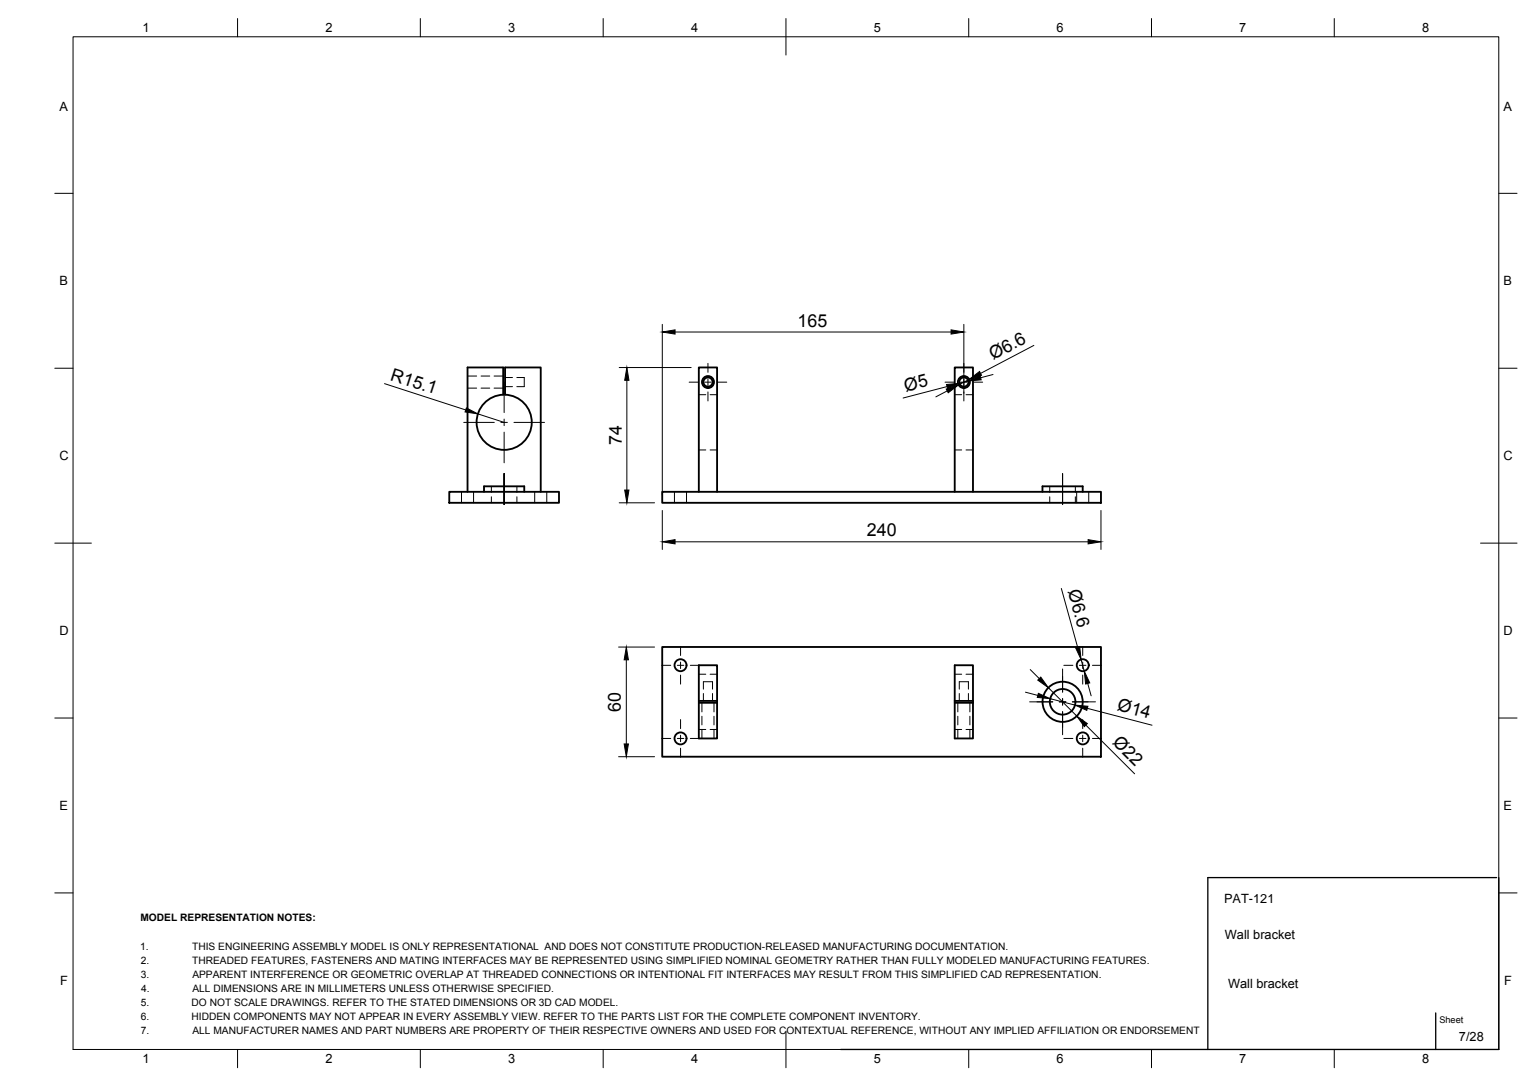
ISO-10303-21;
HEADER;
/* Generated by software containing ST-Developer
 * from STEP Tools, Inc. (www.steptools.com) 
 */

FILE_DESCRIPTION(
/* description */ ('Wall-mounted air drop station'),
/* implementation_level */ '2;1');

FILE_NAME(
/* name */ 'Wall bracket.step',
/* time_stamp */ '2026-10-28T22:16:19-07:00',
/* author */ (''),
/* organization */ (''),
/* preprocessor_version */ 'ST-DEVELOPER v20.2',
/* originating_system */ 'Autodesk Translation Framework v15.17.0.0',
/* authorisation */ '');

FILE_SCHEMA (('AUTOMOTIVE_DESIGN { 1 0 10303 214 3 1 1 }'));
ENDSEC;

DATA;
#10=MECHANICAL_DESIGN_GEOMETRIC_PRESENTATION_REPRESENTATION('',(#346),#10517);
#288=SHAPE_REPRESENTATION_RELATIONSHIP('SRR','None',#10645,#317);
#317=ADVANCED_BREP_SHAPE_REPRESENTATION('',(#375),#10489);
#346=STYLED_ITEM('',(#10853),#375);
#375=MANIFOLD_SOLID_BREP('Body1',#5885);
#407=FACE_BOUND('',#1141,.T.);
#408=FACE_BOUND('',#1146,.T.);
#409=FACE_BOUND('',#1148,.T.);
#410=FACE_BOUND('',#1155,.T.);
#411=FACE_BOUND('',#1161,.T.);
#412=FACE_BOUND('',#1163,.T.);
#413=FACE_BOUND('',#1170,.T.);
#414=FACE_BOUND('',#1174,.T.);
#415=FACE_BOUND('',#1175,.T.);
#416=FACE_BOUND('',#1176,.T.);
#417=FACE_BOUND('',#1177,.T.);
#418=FACE_BOUND('',#1178,.T.);
#419=FACE_BOUND('',#1179,.T.);
#420=FACE_BOUND('',#1180,.T.);
#421=FACE_BOUND('',#1183,.T.);
#422=FACE_BOUND('',#1184,.T.);
#423=FACE_BOUND('',#1185,.T.);
#424=FACE_BOUND('',#1186,.T.);
#425=FACE_BOUND('',#1187,.T.);
#534=PLANE('',#6290);
#535=PLANE('',#6294);
#536=PLANE('',#6298);
#537=PLANE('',#6299);
#538=PLANE('',#6300);
#539=PLANE('',#6304);
#540=PLANE('',#6305);
#541=PLANE('',#6306);
#542=PLANE('',#6307);
#543=PLANE('',#6308);
#544=PLANE('',#6312);
#545=PLANE('',#6316);
#546=PLANE('',#6317);
#547=PLANE('',#6318);
#548=PLANE('',#6322);
#549=PLANE('',#6323);
#550=PLANE('',#6324);
#551=PLANE('',#6325);
#552=PLANE('',#6326);
#553=PLANE('',#6327);
#554=PLANE('',#6328);
#555=PLANE('',#6329);
#556=PLANE('',#6330);
#557=PLANE('',#6331);
#558=PLANE('',#6332);
#771=FACE_OUTER_BOUND('',#1134,.T.);
#772=FACE_OUTER_BOUND('',#1135,.T.);
#773=FACE_OUTER_BOUND('',#1136,.T.);
#774=FACE_OUTER_BOUND('',#1137,.T.);
#775=FACE_OUTER_BOUND('',#1138,.T.);
#776=FACE_OUTER_BOUND('',#1139,.T.);
#777=FACE_OUTER_BOUND('',#1140,.T.);
#778=FACE_OUTER_BOUND('',#1142,.T.);
#779=FACE_OUTER_BOUND('',#1143,.T.);
#780=FACE_OUTER_BOUND('',#1144,.T.);
#781=FACE_OUTER_BOUND('',#1145,.T.);
#782=FACE_OUTER_BOUND('',#1147,.T.);
#783=FACE_OUTER_BOUND('',#1149,.T.);
#784=FACE_OUTER_BOUND('',#1150,.T.);
#785=FACE_OUTER_BOUND('',#1151,.T.);
#786=FACE_OUTER_BOUND('',#1152,.T.);
#787=FACE_OUTER_BOUND('',#1153,.T.);
#788=FACE_OUTER_BOUND('',#1154,.T.);
#789=FACE_OUTER_BOUND('',#1156,.T.);
#790=FACE_OUTER_BOUND('',#1157,.T.);
#791=FACE_OUTER_BOUND('',#1158,.T.);
#792=FACE_OUTER_BOUND('',#1159,.T.);
#793=FACE_OUTER_BOUND('',#1160,.T.);
#794=FACE_OUTER_BOUND('',#1162,.T.);
#795=FACE_OUTER_BOUND('',#1164,.T.);
#796=FACE_OUTER_BOUND('',#1165,.T.);
#797=FACE_OUTER_BOUND('',#1166,.T.);
#798=FACE_OUTER_BOUND('',#1167,.T.);
#799=FACE_OUTER_BOUND('',#1168,.T.);
#800=FACE_OUTER_BOUND('',#1169,.T.);
#801=FACE_OUTER_BOUND('',#1171,.T.);
#802=FACE_OUTER_BOUND('',#1172,.T.);
#803=FACE_OUTER_BOUND('',#1173,.T.);
#804=FACE_OUTER_BOUND('',#1181,.T.);
#805=FACE_OUTER_BOUND('',#1182,.T.);
#806=FACE_OUTER_BOUND('',#1188,.T.);
#807=FACE_OUTER_BOUND('',#1189,.T.);
#1134=EDGE_LOOP('',(#4021,#4022,#4023,#4024));
#1135=EDGE_LOOP('',(#4025,#4026,#4027,#4028));
#1136=EDGE_LOOP('',(#4029,#4030,#4031,#4032));
#1137=EDGE_LOOP('',(#4033,#4034,#4035,#4036));
#1138=EDGE_LOOP('',(#4037,#4038,#4039,#4040));
#1139=EDGE_LOOP('',(#4041,#4042,#4043,#4044));
#1140=EDGE_LOOP('',(#4045));
#1141=EDGE_LOOP('',(#4046));
#1142=EDGE_LOOP('',(#4047,#4048,#4049,#4050));
#1143=EDGE_LOOP('',(#4051));
#1144=EDGE_LOOP('',(#4052,#4053,#4054,#4055));
#1145=EDGE_LOOP('',(#4056,#4057,#4058,#4059));
#1146=EDGE_LOOP('',(#4060));
#1147=EDGE_LOOP('',(#4061,#4062,#4063,#4064));
#1148=EDGE_LOOP('',(#4065));
#1149=EDGE_LOOP('',(#4066,#4067,#4068,#4069,#4070,#4071,#4072,#4073));
#1150=EDGE_LOOP('',(#4074,#4075,#4076,#4077));
#1151=EDGE_LOOP('',(#4078,#4079,#4080,#4081));
#1152=EDGE_LOOP('',(#4082,#4083,#4084,#4085));
#1153=EDGE_LOOP('',(#4086,#4087,#4088,#4089));
#1154=EDGE_LOOP('',(#4090,#4091,#4092,#4093));
#1155=EDGE_LOOP('',(#4094));
#1156=EDGE_LOOP('',(#4095,#4096,#4097,#4098,#4099,#4100,#4101,#4102));
#1157=EDGE_LOOP('',(#4103,#4104,#4105,#4106));
#1158=EDGE_LOOP('',(#4107));
#1159=EDGE_LOOP('',(#4108,#4109,#4110,#4111));
#1160=EDGE_LOOP('',(#4112,#4113,#4114,#4115));
#1161=EDGE_LOOP('',(#4116));
#1162=EDGE_LOOP('',(#4117,#4118,#4119,#4120));
#1163=EDGE_LOOP('',(#4121));
#1164=EDGE_LOOP('',(#4122,#4123,#4124,#4125,#4126,#4127,#4128,#4129));
#1165=EDGE_LOOP('',(#4130,#4131,#4132,#4133));
#1166=EDGE_LOOP('',(#4134,#4135,#4136,#4137));
#1167=EDGE_LOOP('',(#4138,#4139,#4140,#4141));
#1168=EDGE_LOOP('',(#4142,#4143,#4144,#4145));
#1169=EDGE_LOOP('',(#4146,#4147,#4148,#4149));
#1170=EDGE_LOOP('',(#4150));
#1171=EDGE_LOOP('',(#4151,#4152,#4153,#4154,#4155,#4156,#4157,#4158));
#1172=EDGE_LOOP('',(#4159,#4160,#4161,#4162));
#1173=EDGE_LOOP('',(#4163,#4164,#4165,#4166));
#1174=EDGE_LOOP('',(#4167,#4168,#4169,#4170));
#1175=EDGE_LOOP('',(#4171,#4172,#4173,#4174));
#1176=EDGE_LOOP('',(#4175));
#1177=EDGE_LOOP('',(#4176));
#1178=EDGE_LOOP('',(#4177));
#1179=EDGE_LOOP('',(#4178));
#1180=EDGE_LOOP('',(#4179));
#1181=EDGE_LOOP('',(#4180,#4181,#4182,#4183));
#1182=EDGE_LOOP('',(#4184,#4185,#4186,#4187));
#1183=EDGE_LOOP('',(#4188));
#1184=EDGE_LOOP('',(#4189));
#1185=EDGE_LOOP('',(#4190));
#1186=EDGE_LOOP('',(#4191));
#1187=EDGE_LOOP('',(#4192));
#1188=EDGE_LOOP('',(#4193,#4194,#4195,#4196));
#1189=EDGE_LOOP('',(#4197,#4198,#4199,#4200));
#1600=LINE('',#8831,#2064);
#1601=LINE('',#8837,#2065);
#1602=LINE('',#8843,#2066);
#1603=LINE('',#8849,#2067);
#1604=LINE('',#8855,#2068);
#1605=LINE('',#8861,#2069);
#1606=LINE('',#8868,#2070);
#1607=LINE('',#8875,#2071);
#1608=LINE('',#8880,#2072);
#1609=LINE('',#8882,#2073);
#1610=LINE('',#8884,#2074);
#1611=LINE('',#8885,#2075);
#1612=LINE('',#8889,#2076);
#1613=LINE('',#8891,#2077);
#1614=LINE('',#8893,#2078);
#1615=LINE('',#8894,#2079);
#1616=LINE('',#8897,#2080);
#1617=LINE('',#8899,#2081);
#1618=LINE('',#8901,#2082);
#1619=LINE('',#8903,#2083);
#1620=LINE('',#8904,#2084);
#1621=LINE('',#8910,#2085);
#1622=LINE('',#8911,#2086);
#1623=LINE('',#8915,#2087);
#1624=LINE('',#8916,#2088);
#1625=LINE('',#8917,#2089);
#1626=LINE('',#8919,#2090);
#1627=LINE('',#8922,#2091);
#1628=LINE('',#8923,#2092);
#1629=LINE('',#8925,#2093);
#1630=LINE('',#8930,#2094);
#1631=LINE('',#8937,#2095);
#1632=LINE('',#8942,#2096);
#1633=LINE('',#8944,#2097);
#1634=LINE('',#8946,#2098);
#1635=LINE('',#8947,#2099);
#1636=LINE('',#8951,#2100);
#1637=LINE('',#8953,#2101);
#1638=LINE('',#8955,#2102);
#1639=LINE('',#8956,#2103);
#1640=LINE('',#8959,#2104);
#1641=LINE('',#8961,#2105);
#1642=LINE('',#8963,#2106);
#1643=LINE('',#8965,#2107);
#1644=LINE('',#8966,#2108);
#1645=LINE('',#8972,#2109);
#1646=LINE('',#8973,#2110);
#1647=LINE('',#8977,#2111);
#1648=LINE('',#8978,#2112);
#1649=LINE('',#8979,#2113);
#1650=LINE('',#8981,#2114);
#1651=LINE('',#8984,#2115);
#1652=LINE('',#8985,#2116);
#1653=LINE('',#8987,#2117);
#1654=LINE('',#8991,#2118);
#1655=LINE('',#8993,#2119);
#1656=LINE('',#8995,#2120);
#1657=LINE('',#8996,#2121);
#1658=LINE('',#8999,#2122);
#1659=LINE('',#9001,#2123);
#1660=LINE('',#9002,#2124);
#1661=LINE('',#9005,#2125);
#1662=LINE('',#9007,#2126);
#1663=LINE('',#9008,#2127);
#1664=LINE('',#9010,#2128);
#1665=LINE('',#9011,#2129);
#2064=VECTOR('',#7010,0.33);
#2065=VECTOR('',#7017,0.33);
#2066=VECTOR('',#7024,0.33);
#2067=VECTOR('',#7031,0.33);
#2068=VECTOR('',#7038,0.7);
#2069=VECTOR('',#7045,1.1);
#2070=VECTOR('',#7054,0.25);
#2071=VECTOR('',#7063,0.33);
#2072=VECTOR('',#7068,1.);
#2073=VECTOR('',#7069,1.);
#2074=VECTOR('',#7070,1.);
#2075=VECTOR('',#7071,1.);
#2076=VECTOR('',#7074,1.);
#2077=VECTOR('',#7075,1.);
#2078=VECTOR('',#7076,1.);
#2079=VECTOR('',#7077,1.);
#2080=VECTOR('',#7080,1.);
#2081=VECTOR('',#7081,1.);
#2082=VECTOR('',#7082,1.);
#2083=VECTOR('',#7083,1.);
#2084=VECTOR('',#7084,1.);
#2085=VECTOR('',#7093,1.);
#2086=VECTOR('',#7094,1.);
#2087=VECTOR('',#7097,1.);
#2088=VECTOR('',#7098,1.);
#2089=VECTOR('',#7099,1.);
#2090=VECTOR('',#7102,1.);
#2091=VECTOR('',#7105,1.);
#2092=VECTOR('',#7106,1.);
#2093=VECTOR('',#7109,1.);
#2094=VECTOR('',#7114,0.25);
#2095=VECTOR('',#7123,0.33);
#2096=VECTOR('',#7128,1.);
#2097=VECTOR('',#7129,1.);
#2098=VECTOR('',#7130,1.);
#2099=VECTOR('',#7131,1.);
#2100=VECTOR('',#7134,1.);
#2101=VECTOR('',#7135,1.);
#2102=VECTOR('',#7136,1.);
#2103=VECTOR('',#7137,1.);
#2104=VECTOR('',#7140,1.);
#2105=VECTOR('',#7141,1.);
#2106=VECTOR('',#7142,1.);
#2107=VECTOR('',#7143,1.);
#2108=VECTOR('',#7144,1.);
#2109=VECTOR('',#7153,1.);
#2110=VECTOR('',#7154,1.);
#2111=VECTOR('',#7157,1.);
#2112=VECTOR('',#7158,1.);
#2113=VECTOR('',#7159,1.);
#2114=VECTOR('',#7162,1.);
#2115=VECTOR('',#7165,1.);
#2116=VECTOR('',#7166,1.);
#2117=VECTOR('',#7169,1.);
#2118=VECTOR('',#7172,1.);
#2119=VECTOR('',#7173,1.);
#2120=VECTOR('',#7174,1.);
#2121=VECTOR('',#7175,1.);
#2122=VECTOR('',#7178,1.);
#2123=VECTOR('',#7179,1.);
#2124=VECTOR('',#7180,1.);
#2125=VECTOR('',#7183,1.);
#2126=VECTOR('',#7184,1.);
#2127=VECTOR('',#7185,1.);
#2128=VECTOR('',#7188,1.);
#2129=VECTOR('',#7189,1.);
#2536=CIRCLE('',#6273,0.33);
#2537=CIRCLE('',#6274,0.33);
#2538=CIRCLE('',#6276,0.33);
#2539=CIRCLE('',#6277,0.33);
#2540=CIRCLE('',#6279,0.33);
#2541=CIRCLE('',#6280,0.33);
#2542=CIRCLE('',#6282,0.33);
#2543=CIRCLE('',#6283,0.33);
#2544=CIRCLE('',#6285,0.7);
#2545=CIRCLE('',#6286,0.7);
#2546=CIRCLE('',#6288,1.1);
#2547=CIRCLE('',#6289,1.1);
#2548=CIRCLE('',#6292,0.25);
#2549=CIRCLE('',#6293,0.25);
#2550=CIRCLE('',#6296,0.33);
#2551=CIRCLE('',#6297,0.33);
#2552=CIRCLE('',#6301,1.51);
#2553=CIRCLE('',#6303,1.51);
#2554=CIRCLE('',#6310,0.25);
#2555=CIRCLE('',#6311,0.25);
#2556=CIRCLE('',#6314,0.33);
#2557=CIRCLE('',#6315,0.33);
#2558=CIRCLE('',#6319,1.51);
#2559=CIRCLE('',#6321,1.51);
#2781=VERTEX_POINT('',#8828);
#2782=VERTEX_POINT('',#8830);
#2783=VERTEX_POINT('',#8834);
#2784=VERTEX_POINT('',#8836);
#2785=VERTEX_POINT('',#8840);
#2786=VERTEX_POINT('',#8842);
#2787=VERTEX_POINT('',#8846);
#2788=VERTEX_POINT('',#8848);
#2789=VERTEX_POINT('',#8852);
#2790=VERTEX_POINT('',#8854);
#2791=VERTEX_POINT('',#8858);
#2792=VERTEX_POINT('',#8860);
#2793=VERTEX_POINT('',#8865);
#2794=VERTEX_POINT('',#8867);
#2795=VERTEX_POINT('',#8872);
#2796=VERTEX_POINT('',#8874);
#2797=VERTEX_POINT('',#8878);
#2798=VERTEX_POINT('',#8879);
#2799=VERTEX_POINT('',#8881);
#2800=VERTEX_POINT('',#8883);
#2801=VERTEX_POINT('',#8887);
#2802=VERTEX_POINT('',#8888);
#2803=VERTEX_POINT('',#8890);
#2804=VERTEX_POINT('',#8892);
#2805=VERTEX_POINT('',#8896);
#2806=VERTEX_POINT('',#8898);
#2807=VERTEX_POINT('',#8900);
#2808=VERTEX_POINT('',#8902);
#2809=VERTEX_POINT('',#8909);
#2810=VERTEX_POINT('',#8913);
#2811=VERTEX_POINT('',#8914);
#2812=VERTEX_POINT('',#8921);
#2813=VERTEX_POINT('',#8927);
#2814=VERTEX_POINT('',#8929);
#2815=VERTEX_POINT('',#8934);
#2816=VERTEX_POINT('',#8936);
#2817=VERTEX_POINT('',#8940);
#2818=VERTEX_POINT('',#8941);
#2819=VERTEX_POINT('',#8943);
#2820=VERTEX_POINT('',#8945);
#2821=VERTEX_POINT('',#8949);
#2822=VERTEX_POINT('',#8950);
#2823=VERTEX_POINT('',#8952);
#2824=VERTEX_POINT('',#8954);
#2825=VERTEX_POINT('',#8958);
#2826=VERTEX_POINT('',#8960);
#2827=VERTEX_POINT('',#8962);
#2828=VERTEX_POINT('',#8964);
#2829=VERTEX_POINT('',#8971);
#2830=VERTEX_POINT('',#8975);
#2831=VERTEX_POINT('',#8976);
#2832=VERTEX_POINT('',#8983);
#2833=VERTEX_POINT('',#8989);
#2834=VERTEX_POINT('',#8990);
#2835=VERTEX_POINT('',#8992);
#2836=VERTEX_POINT('',#8994);
#2837=VERTEX_POINT('',#8998);
#2838=VERTEX_POINT('',#9000);
#2839=VERTEX_POINT('',#9004);
#2840=VERTEX_POINT('',#9006);
#3268=EDGE_CURVE('',#2781,#2781,#2536,.T.);
#3269=EDGE_CURVE('',#2781,#2782,#1600,.T.);
#3270=EDGE_CURVE('',#2782,#2782,#2537,.T.);
#3271=EDGE_CURVE('',#2783,#2783,#2538,.T.);
#3272=EDGE_CURVE('',#2783,#2784,#1601,.T.);
#3273=EDGE_CURVE('',#2784,#2784,#2539,.T.);
#3274=EDGE_CURVE('',#2785,#2785,#2540,.T.);
#3275=EDGE_CURVE('',#2785,#2786,#1602,.T.);
#3276=EDGE_CURVE('',#2786,#2786,#2541,.T.);
#3277=EDGE_CURVE('',#2787,#2787,#2542,.T.);
#3278=EDGE_CURVE('',#2787,#2788,#1603,.T.);
#3279=EDGE_CURVE('',#2788,#2788,#2543,.T.);
#3280=EDGE_CURVE('',#2789,#2789,#2544,.T.);
#3281=EDGE_CURVE('',#2789,#2790,#1604,.T.);
#3282=EDGE_CURVE('',#2790,#2790,#2545,.T.);
#3283=EDGE_CURVE('',#2791,#2791,#2546,.T.);
#3284=EDGE_CURVE('',#2791,#2792,#1605,.T.);
#3285=EDGE_CURVE('',#2792,#2792,#2547,.T.);
#3286=EDGE_CURVE('',#2793,#2793,#2548,.T.);
#3287=EDGE_CURVE('',#2793,#2794,#1606,.T.);
#3288=EDGE_CURVE('',#2794,#2794,#2549,.T.);
#3289=EDGE_CURVE('',#2795,#2795,#2550,.T.);
#3290=EDGE_CURVE('',#2795,#2796,#1607,.T.);
#3291=EDGE_CURVE('',#2796,#2796,#2551,.T.);
#3292=EDGE_CURVE('',#2797,#2798,#1608,.T.);
#3293=EDGE_CURVE('',#2799,#2797,#1609,.T.);
#3294=EDGE_CURVE('',#2800,#2799,#1610,.T.);
#3295=EDGE_CURVE('',#2798,#2800,#1611,.T.);
#3296=EDGE_CURVE('',#2801,#2802,#1612,.T.);
#3297=EDGE_CURVE('',#2803,#2801,#1613,.T.);
#3298=EDGE_CURVE('',#2804,#2803,#1614,.T.);
#3299=EDGE_CURVE('',#2802,#2804,#1615,.T.);
#3300=EDGE_CURVE('',#2797,#2805,#1616,.T.);
#3301=EDGE_CURVE('',#2805,#2806,#1617,.T.);
#3302=EDGE_CURVE('',#2807,#2806,#1618,.T.);
#3303=EDGE_CURVE('',#2807,#2808,#1619,.T.);
#3304=EDGE_CURVE('',#2808,#2802,#1620,.T.);
#3305=EDGE_CURVE('',#2804,#2799,#2552,.T.);
#3306=EDGE_CURVE('',#2800,#2803,#2553,.T.);
#3307=EDGE_CURVE('',#2809,#2808,#1621,.T.);
#3308=EDGE_CURVE('',#2801,#2809,#1622,.T.);
#3309=EDGE_CURVE('',#2810,#2811,#1623,.T.);
#3310=EDGE_CURVE('',#2806,#2810,#1624,.T.);
#3311=EDGE_CURVE('',#2811,#2805,#1625,.T.);
#3312=EDGE_CURVE('',#2811,#2798,#1626,.T.);
#3313=EDGE_CURVE('',#2809,#2812,#1627,.T.);
#3314=EDGE_CURVE('',#2812,#2807,#1628,.T.);
#3315=EDGE_CURVE('',#2810,#2812,#1629,.T.);
#3316=EDGE_CURVE('',#2813,#2813,#2554,.T.);
#3317=EDGE_CURVE('',#2813,#2814,#1630,.T.);
#3318=EDGE_CURVE('',#2814,#2814,#2555,.T.);
#3319=EDGE_CURVE('',#2815,#2815,#2556,.T.);
#3320=EDGE_CURVE('',#2815,#2816,#1631,.T.);
#3321=EDGE_CURVE('',#2816,#2816,#2557,.T.);
#3322=EDGE_CURVE('',#2817,#2818,#1632,.T.);
#3323=EDGE_CURVE('',#2819,#2817,#1633,.T.);
#3324=EDGE_CURVE('',#2820,#2819,#1634,.T.);
#3325=EDGE_CURVE('',#2818,#2820,#1635,.T.);
#3326=EDGE_CURVE('',#2821,#2822,#1636,.T.);
#3327=EDGE_CURVE('',#2823,#2821,#1637,.T.);
#3328=EDGE_CURVE('',#2824,#2823,#1638,.T.);
#3329=EDGE_CURVE('',#2822,#2824,#1639,.T.);
#3330=EDGE_CURVE('',#2817,#2825,#1640,.T.);
#3331=EDGE_CURVE('',#2825,#2826,#1641,.T.);
#3332=EDGE_CURVE('',#2827,#2826,#1642,.T.);
#3333=EDGE_CURVE('',#2827,#2828,#1643,.T.);
#3334=EDGE_CURVE('',#2828,#2822,#1644,.T.);
#3335=EDGE_CURVE('',#2824,#2819,#2558,.T.);
#3336=EDGE_CURVE('',#2820,#2823,#2559,.T.);
#3337=EDGE_CURVE('',#2829,#2828,#1645,.T.);
#3338=EDGE_CURVE('',#2821,#2829,#1646,.T.);
#3339=EDGE_CURVE('',#2830,#2831,#1647,.T.);
#3340=EDGE_CURVE('',#2826,#2830,#1648,.T.);
#3341=EDGE_CURVE('',#2831,#2825,#1649,.T.);
#3342=EDGE_CURVE('',#2831,#2818,#1650,.T.);
#3343=EDGE_CURVE('',#2829,#2832,#1651,.T.);
#3344=EDGE_CURVE('',#2832,#2827,#1652,.T.);
#3345=EDGE_CURVE('',#2830,#2832,#1653,.T.);
#3346=EDGE_CURVE('',#2833,#2834,#1654,.T.);
#3347=EDGE_CURVE('',#2834,#2835,#1655,.T.);
#3348=EDGE_CURVE('',#2836,#2835,#1656,.T.);
#3349=EDGE_CURVE('',#2833,#2836,#1657,.T.);
#3350=EDGE_CURVE('',#2837,#2833,#1658,.T.);
#3351=EDGE_CURVE('',#2838,#2836,#1659,.T.);
#3352=EDGE_CURVE('',#2837,#2838,#1660,.T.);
#3353=EDGE_CURVE('',#2839,#2837,#1661,.T.);
#3354=EDGE_CURVE('',#2840,#2838,#1662,.T.);
#3355=EDGE_CURVE('',#2839,#2840,#1663,.T.);
#3356=EDGE_CURVE('',#2834,#2839,#1664,.T.);
#3357=EDGE_CURVE('',#2835,#2840,#1665,.T.);
#4021=ORIENTED_EDGE('',*,*,#3268,.F.);
#4022=ORIENTED_EDGE('',*,*,#3269,.T.);
#4023=ORIENTED_EDGE('',*,*,#3270,.F.);
#4024=ORIENTED_EDGE('',*,*,#3269,.F.);
#4025=ORIENTED_EDGE('',*,*,#3271,.F.);
#4026=ORIENTED_EDGE('',*,*,#3272,.T.);
#4027=ORIENTED_EDGE('',*,*,#3273,.F.);
#4028=ORIENTED_EDGE('',*,*,#3272,.F.);
#4029=ORIENTED_EDGE('',*,*,#3274,.F.);
#4030=ORIENTED_EDGE('',*,*,#3275,.T.);
#4031=ORIENTED_EDGE('',*,*,#3276,.F.);
#4032=ORIENTED_EDGE('',*,*,#3275,.F.);
#4033=ORIENTED_EDGE('',*,*,#3277,.F.);
#4034=ORIENTED_EDGE('',*,*,#3278,.T.);
#4035=ORIENTED_EDGE('',*,*,#3279,.F.);
#4036=ORIENTED_EDGE('',*,*,#3278,.F.);
#4037=ORIENTED_EDGE('',*,*,#3280,.F.);
#4038=ORIENTED_EDGE('',*,*,#3281,.T.);
#4039=ORIENTED_EDGE('',*,*,#3282,.F.);
#4040=ORIENTED_EDGE('',*,*,#3281,.F.);
#4041=ORIENTED_EDGE('',*,*,#3283,.F.);
#4042=ORIENTED_EDGE('',*,*,#3284,.T.);
#4043=ORIENTED_EDGE('',*,*,#3285,.F.);
#4044=ORIENTED_EDGE('',*,*,#3284,.F.);
#4045=ORIENTED_EDGE('',*,*,#3283,.T.);
#4046=ORIENTED_EDGE('',*,*,#3282,.T.);
#4047=ORIENTED_EDGE('',*,*,#3286,.F.);
#4048=ORIENTED_EDGE('',*,*,#3287,.T.);
#4049=ORIENTED_EDGE('',*,*,#3288,.F.);
#4050=ORIENTED_EDGE('',*,*,#3287,.F.);
#4051=ORIENTED_EDGE('',*,*,#3286,.T.);
#4052=ORIENTED_EDGE('',*,*,#3289,.F.);
#4053=ORIENTED_EDGE('',*,*,#3290,.T.);
#4054=ORIENTED_EDGE('',*,*,#3291,.F.);
#4055=ORIENTED_EDGE('',*,*,#3290,.F.);
#4056=ORIENTED_EDGE('',*,*,#3292,.F.);
#4057=ORIENTED_EDGE('',*,*,#3293,.F.);
#4058=ORIENTED_EDGE('',*,*,#3294,.F.);
#4059=ORIENTED_EDGE('',*,*,#3295,.F.);
#4060=ORIENTED_EDGE('',*,*,#3288,.T.);
#4061=ORIENTED_EDGE('',*,*,#3296,.F.);
#4062=ORIENTED_EDGE('',*,*,#3297,.F.);
#4063=ORIENTED_EDGE('',*,*,#3298,.F.);
#4064=ORIENTED_EDGE('',*,*,#3299,.F.);
#4065=ORIENTED_EDGE('',*,*,#3289,.T.);
#4066=ORIENTED_EDGE('',*,*,#3293,.T.);
#4067=ORIENTED_EDGE('',*,*,#3300,.T.);
#4068=ORIENTED_EDGE('',*,*,#3301,.T.);
#4069=ORIENTED_EDGE('',*,*,#3302,.F.);
#4070=ORIENTED_EDGE('',*,*,#3303,.T.);
#4071=ORIENTED_EDGE('',*,*,#3304,.T.);
#4072=ORIENTED_EDGE('',*,*,#3299,.T.);
#4073=ORIENTED_EDGE('',*,*,#3305,.T.);
#4074=ORIENTED_EDGE('',*,*,#3294,.T.);
#4075=ORIENTED_EDGE('',*,*,#3305,.F.);
#4076=ORIENTED_EDGE('',*,*,#3298,.T.);
#4077=ORIENTED_EDGE('',*,*,#3306,.F.);
#4078=ORIENTED_EDGE('',*,*,#3296,.T.);
#4079=ORIENTED_EDGE('',*,*,#3304,.F.);
#4080=ORIENTED_EDGE('',*,*,#3307,.F.);
#4081=ORIENTED_EDGE('',*,*,#3308,.F.);
#4082=ORIENTED_EDGE('',*,*,#3309,.F.);
#4083=ORIENTED_EDGE('',*,*,#3310,.F.);
#4084=ORIENTED_EDGE('',*,*,#3301,.F.);
#4085=ORIENTED_EDGE('',*,*,#3311,.F.);
#4086=ORIENTED_EDGE('',*,*,#3292,.T.);
#4087=ORIENTED_EDGE('',*,*,#3312,.F.);
#4088=ORIENTED_EDGE('',*,*,#3311,.T.);
#4089=ORIENTED_EDGE('',*,*,#3300,.F.);
#4090=ORIENTED_EDGE('',*,*,#3313,.F.);
#4091=ORIENTED_EDGE('',*,*,#3307,.T.);
#4092=ORIENTED_EDGE('',*,*,#3303,.F.);
#4093=ORIENTED_EDGE('',*,*,#3314,.F.);
#4094=ORIENTED_EDGE('',*,*,#3291,.T.);
#4095=ORIENTED_EDGE('',*,*,#3295,.T.);
#4096=ORIENTED_EDGE('',*,*,#3306,.T.);
#4097=ORIENTED_EDGE('',*,*,#3297,.T.);
#4098=ORIENTED_EDGE('',*,*,#3308,.T.);
#4099=ORIENTED_EDGE('',*,*,#3313,.T.);
#4100=ORIENTED_EDGE('',*,*,#3315,.F.);
#4101=ORIENTED_EDGE('',*,*,#3309,.T.);
#4102=ORIENTED_EDGE('',*,*,#3312,.T.);
#4103=ORIENTED_EDGE('',*,*,#3316,.F.);
#4104=ORIENTED_EDGE('',*,*,#3317,.T.);
#4105=ORIENTED_EDGE('',*,*,#3318,.F.);
#4106=ORIENTED_EDGE('',*,*,#3317,.F.);
#4107=ORIENTED_EDGE('',*,*,#3316,.T.);
#4108=ORIENTED_EDGE('',*,*,#3319,.F.);
#4109=ORIENTED_EDGE('',*,*,#3320,.T.);
#4110=ORIENTED_EDGE('',*,*,#3321,.F.);
#4111=ORIENTED_EDGE('',*,*,#3320,.F.);
#4112=ORIENTED_EDGE('',*,*,#3322,.F.);
#4113=ORIENTED_EDGE('',*,*,#3323,.F.);
#4114=ORIENTED_EDGE('',*,*,#3324,.F.);
#4115=ORIENTED_EDGE('',*,*,#3325,.F.);
#4116=ORIENTED_EDGE('',*,*,#3318,.T.);
#4117=ORIENTED_EDGE('',*,*,#3326,.F.);
#4118=ORIENTED_EDGE('',*,*,#3327,.F.);
#4119=ORIENTED_EDGE('',*,*,#3328,.F.);
#4120=ORIENTED_EDGE('',*,*,#3329,.F.);
#4121=ORIENTED_EDGE('',*,*,#3319,.T.);
#4122=ORIENTED_EDGE('',*,*,#3323,.T.);
#4123=ORIENTED_EDGE('',*,*,#3330,.T.);
#4124=ORIENTED_EDGE('',*,*,#3331,.T.);
#4125=ORIENTED_EDGE('',*,*,#3332,.F.);
#4126=ORIENTED_EDGE('',*,*,#3333,.T.);
#4127=ORIENTED_EDGE('',*,*,#3334,.T.);
#4128=ORIENTED_EDGE('',*,*,#3329,.T.);
#4129=ORIENTED_EDGE('',*,*,#3335,.T.);
#4130=ORIENTED_EDGE('',*,*,#3324,.T.);
#4131=ORIENTED_EDGE('',*,*,#3335,.F.);
#4132=ORIENTED_EDGE('',*,*,#3328,.T.);
#4133=ORIENTED_EDGE('',*,*,#3336,.F.);
#4134=ORIENTED_EDGE('',*,*,#3326,.T.);
#4135=ORIENTED_EDGE('',*,*,#3334,.F.);
#4136=ORIENTED_EDGE('',*,*,#3337,.F.);
#4137=ORIENTED_EDGE('',*,*,#3338,.F.);
#4138=ORIENTED_EDGE('',*,*,#3339,.F.);
#4139=ORIENTED_EDGE('',*,*,#3340,.F.);
#4140=ORIENTED_EDGE('',*,*,#3331,.F.);
#4141=ORIENTED_EDGE('',*,*,#3341,.F.);
#4142=ORIENTED_EDGE('',*,*,#3322,.T.);
#4143=ORIENTED_EDGE('',*,*,#3342,.F.);
#4144=ORIENTED_EDGE('',*,*,#3341,.T.);
#4145=ORIENTED_EDGE('',*,*,#3330,.F.);
#4146=ORIENTED_EDGE('',*,*,#3343,.F.);
#4147=ORIENTED_EDGE('',*,*,#3337,.T.);
#4148=ORIENTED_EDGE('',*,*,#3333,.F.);
#4149=ORIENTED_EDGE('',*,*,#3344,.F.);
#4150=ORIENTED_EDGE('',*,*,#3321,.T.);
#4151=ORIENTED_EDGE('',*,*,#3325,.T.);
#4152=ORIENTED_EDGE('',*,*,#3336,.T.);
#4153=ORIENTED_EDGE('',*,*,#3327,.T.);
#4154=ORIENTED_EDGE('',*,*,#3338,.T.);
#4155=ORIENTED_EDGE('',*,*,#3343,.T.);
#4156=ORIENTED_EDGE('',*,*,#3345,.F.);
#4157=ORIENTED_EDGE('',*,*,#3339,.T.);
#4158=ORIENTED_EDGE('',*,*,#3342,.T.);
#4159=ORIENTED_EDGE('',*,*,#3346,.T.);
#4160=ORIENTED_EDGE('',*,*,#3347,.T.);
#4161=ORIENTED_EDGE('',*,*,#3348,.F.);
#4162=ORIENTED_EDGE('',*,*,#3349,.F.);
#4163=ORIENTED_EDGE('',*,*,#3350,.T.);
#4164=ORIENTED_EDGE('',*,*,#3349,.T.);
#4165=ORIENTED_EDGE('',*,*,#3351,.F.);
#4166=ORIENTED_EDGE('',*,*,#3352,.F.);
#4167=ORIENTED_EDGE('',*,*,#3344,.T.);
#4168=ORIENTED_EDGE('',*,*,#3332,.T.);
#4169=ORIENTED_EDGE('',*,*,#3340,.T.);
#4170=ORIENTED_EDGE('',*,*,#3345,.T.);
#4171=ORIENTED_EDGE('',*,*,#3314,.T.);
#4172=ORIENTED_EDGE('',*,*,#3302,.T.);
#4173=ORIENTED_EDGE('',*,*,#3310,.T.);
#4174=ORIENTED_EDGE('',*,*,#3315,.T.);
#4175=ORIENTED_EDGE('',*,*,#3285,.T.);
#4176=ORIENTED_EDGE('',*,*,#3279,.T.);
#4177=ORIENTED_EDGE('',*,*,#3276,.T.);
#4178=ORIENTED_EDGE('',*,*,#3273,.T.);
#4179=ORIENTED_EDGE('',*,*,#3270,.T.);
#4180=ORIENTED_EDGE('',*,*,#3353,.T.);
#4181=ORIENTED_EDGE('',*,*,#3352,.T.);
#4182=ORIENTED_EDGE('',*,*,#3354,.F.);
#4183=ORIENTED_EDGE('',*,*,#3355,.F.);
#4184=ORIENTED_EDGE('',*,*,#3356,.T.);
#4185=ORIENTED_EDGE('',*,*,#3355,.T.);
#4186=ORIENTED_EDGE('',*,*,#3357,.F.);
#4187=ORIENTED_EDGE('',*,*,#3347,.F.);
#4188=ORIENTED_EDGE('',*,*,#3280,.T.);
#4189=ORIENTED_EDGE('',*,*,#3277,.T.);
#4190=ORIENTED_EDGE('',*,*,#3274,.T.);
#4191=ORIENTED_EDGE('',*,*,#3271,.T.);
#4192=ORIENTED_EDGE('',*,*,#3268,.T.);
#4193=ORIENTED_EDGE('',*,*,#3357,.T.);
#4194=ORIENTED_EDGE('',*,*,#3354,.T.);
#4195=ORIENTED_EDGE('',*,*,#3351,.T.);
#4196=ORIENTED_EDGE('',*,*,#3348,.T.);
#4197=ORIENTED_EDGE('',*,*,#3356,.F.);
#4198=ORIENTED_EDGE('',*,*,#3346,.F.);
#4199=ORIENTED_EDGE('',*,*,#3350,.F.);
#4200=ORIENTED_EDGE('',*,*,#3353,.F.);
#5439=CYLINDRICAL_SURFACE('',#6272,0.33);
#5440=CYLINDRICAL_SURFACE('',#6275,0.33);
#5441=CYLINDRICAL_SURFACE('',#6278,0.33);
#5442=CYLINDRICAL_SURFACE('',#6281,0.33);
#5443=CYLINDRICAL_SURFACE('',#6284,0.7);
#5444=CYLINDRICAL_SURFACE('',#6287,1.1);
#5445=CYLINDRICAL_SURFACE('',#6291,0.25);
#5446=CYLINDRICAL_SURFACE('',#6295,0.33);
#5447=CYLINDRICAL_SURFACE('',#6302,1.51);
#5448=CYLINDRICAL_SURFACE('',#6309,0.25);
#5449=CYLINDRICAL_SURFACE('',#6313,0.33);
#5450=CYLINDRICAL_SURFACE('',#6320,1.51);
#5544=ADVANCED_FACE('',(#771),#5439,.F.);
#5545=ADVANCED_FACE('',(#772),#5440,.F.);
#5546=ADVANCED_FACE('',(#773),#5441,.F.);
#5547=ADVANCED_FACE('',(#774),#5442,.F.);
#5548=ADVANCED_FACE('',(#775),#5443,.F.);
#5549=ADVANCED_FACE('',(#776),#5444,.T.);
#5550=ADVANCED_FACE('',(#777,#407),#534,.T.);
#5551=ADVANCED_FACE('',(#778),#5445,.F.);
#5552=ADVANCED_FACE('',(#779),#535,.T.);
#5553=ADVANCED_FACE('',(#780),#5446,.F.);
#5554=ADVANCED_FACE('',(#781,#408),#536,.F.);
#5555=ADVANCED_FACE('',(#782,#409),#537,.F.);
#5556=ADVANCED_FACE('',(#783),#538,.T.);
#5557=ADVANCED_FACE('',(#784),#5447,.F.);
#5558=ADVANCED_FACE('',(#785),#539,.T.);
#5559=ADVANCED_FACE('',(#786),#540,.T.);
#5560=ADVANCED_FACE('',(#787),#541,.T.);
#5561=ADVANCED_FACE('',(#788,#410),#542,.T.);
#5562=ADVANCED_FACE('',(#789),#543,.F.);
#5563=ADVANCED_FACE('',(#790),#5448,.F.);
#5564=ADVANCED_FACE('',(#791),#544,.T.);
#5565=ADVANCED_FACE('',(#792),#5449,.F.);
#5566=ADVANCED_FACE('',(#793,#411),#545,.F.);
#5567=ADVANCED_FACE('',(#794,#412),#546,.F.);
#5568=ADVANCED_FACE('',(#795),#547,.T.);
#5569=ADVANCED_FACE('',(#796),#5450,.F.);
#5570=ADVANCED_FACE('',(#797),#548,.T.);
#5571=ADVANCED_FACE('',(#798),#549,.T.);
#5572=ADVANCED_FACE('',(#799),#550,.T.);
#5573=ADVANCED_FACE('',(#800,#413),#551,.T.);
#5574=ADVANCED_FACE('',(#801),#552,.F.);
#5575=ADVANCED_FACE('',(#802),#553,.T.);
#5576=ADVANCED_FACE('',(#803,#414,#415,#416,#417,#418,#419,#420),#554,.T.);
#5577=ADVANCED_FACE('',(#804),#555,.T.);
#5578=ADVANCED_FACE('',(#805,#421,#422,#423,#424,#425),#556,.T.);
#5579=ADVANCED_FACE('',(#806),#557,.T.);
#5580=ADVANCED_FACE('',(#807),#558,.F.);
#5885=CLOSED_SHELL('',(#5544,#5545,#5546,#5547,#5548,#5549,#5550,#5551,
#5552,#5553,#5554,#5555,#5556,#5557,#5558,#5559,#5560,#5561,#5562,#5563,
#5564,#5565,#5566,#5567,#5568,#5569,#5570,#5571,#5572,#5573,#5574,#5575,
#5576,#5577,#5578,#5579,#5580));
#6271=AXIS2_PLACEMENT_3D('',#8826,#7004,#7005);
#6272=AXIS2_PLACEMENT_3D('',#8827,#7006,#7007);
#6273=AXIS2_PLACEMENT_3D('',#8829,#7008,#7009);
#6274=AXIS2_PLACEMENT_3D('',#8832,#7011,#7012);
#6275=AXIS2_PLACEMENT_3D('',#8833,#7013,#7014);
#6276=AXIS2_PLACEMENT_3D('',#8835,#7015,#7016);
#6277=AXIS2_PLACEMENT_3D('',#8838,#7018,#7019);
#6278=AXIS2_PLACEMENT_3D('',#8839,#7020,#7021);
#6279=AXIS2_PLACEMENT_3D('',#8841,#7022,#7023);
#6280=AXIS2_PLACEMENT_3D('',#8844,#7025,#7026);
#6281=AXIS2_PLACEMENT_3D('',#8845,#7027,#7028);
#6282=AXIS2_PLACEMENT_3D('',#8847,#7029,#7030);
#6283=AXIS2_PLACEMENT_3D('',#8850,#7032,#7033);
#6284=AXIS2_PLACEMENT_3D('',#8851,#7034,#7035);
#6285=AXIS2_PLACEMENT_3D('',#8853,#7036,#7037);
#6286=AXIS2_PLACEMENT_3D('',#8856,#7039,#7040);
#6287=AXIS2_PLACEMENT_3D('',#8857,#7041,#7042);
#6288=AXIS2_PLACEMENT_3D('',#8859,#7043,#7044);
#6289=AXIS2_PLACEMENT_3D('',#8862,#7046,#7047);
#6290=AXIS2_PLACEMENT_3D('',#8863,#7048,#7049);
#6291=AXIS2_PLACEMENT_3D('',#8864,#7050,#7051);
#6292=AXIS2_PLACEMENT_3D('',#8866,#7052,#7053);
#6293=AXIS2_PLACEMENT_3D('',#8869,#7055,#7056);
#6294=AXIS2_PLACEMENT_3D('',#8870,#7057,#7058);
#6295=AXIS2_PLACEMENT_3D('',#8871,#7059,#7060);
#6296=AXIS2_PLACEMENT_3D('',#8873,#7061,#7062);
#6297=AXIS2_PLACEMENT_3D('',#8876,#7064,#7065);
#6298=AXIS2_PLACEMENT_3D('',#8877,#7066,#7067);
#6299=AXIS2_PLACEMENT_3D('',#8886,#7072,#7073);
#6300=AXIS2_PLACEMENT_3D('',#8895,#7078,#7079);
#6301=AXIS2_PLACEMENT_3D('',#8905,#7085,#7086);
#6302=AXIS2_PLACEMENT_3D('',#8906,#7087,#7088);
#6303=AXIS2_PLACEMENT_3D('',#8907,#7089,#7090);
#6304=AXIS2_PLACEMENT_3D('',#8908,#7091,#7092);
#6305=AXIS2_PLACEMENT_3D('',#8912,#7095,#7096);
#6306=AXIS2_PLACEMENT_3D('',#8918,#7100,#7101);
#6307=AXIS2_PLACEMENT_3D('',#8920,#7103,#7104);
#6308=AXIS2_PLACEMENT_3D('',#8924,#7107,#7108);
#6309=AXIS2_PLACEMENT_3D('',#8926,#7110,#7111);
#6310=AXIS2_PLACEMENT_3D('',#8928,#7112,#7113);
#6311=AXIS2_PLACEMENT_3D('',#8931,#7115,#7116);
#6312=AXIS2_PLACEMENT_3D('',#8932,#7117,#7118);
#6313=AXIS2_PLACEMENT_3D('',#8933,#7119,#7120);
#6314=AXIS2_PLACEMENT_3D('',#8935,#7121,#7122);
#6315=AXIS2_PLACEMENT_3D('',#8938,#7124,#7125);
#6316=AXIS2_PLACEMENT_3D('',#8939,#7126,#7127);
#6317=AXIS2_PLACEMENT_3D('',#8948,#7132,#7133);
#6318=AXIS2_PLACEMENT_3D('',#8957,#7138,#7139);
#6319=AXIS2_PLACEMENT_3D('',#8967,#7145,#7146);
#6320=AXIS2_PLACEMENT_3D('',#8968,#7147,#7148);
#6321=AXIS2_PLACEMENT_3D('',#8969,#7149,#7150);
#6322=AXIS2_PLACEMENT_3D('',#8970,#7151,#7152);
#6323=AXIS2_PLACEMENT_3D('',#8974,#7155,#7156);
#6324=AXIS2_PLACEMENT_3D('',#8980,#7160,#7161);
#6325=AXIS2_PLACEMENT_3D('',#8982,#7163,#7164);
#6326=AXIS2_PLACEMENT_3D('',#8986,#7167,#7168);
#6327=AXIS2_PLACEMENT_3D('',#8988,#7170,#7171);
#6328=AXIS2_PLACEMENT_3D('',#8997,#7176,#7177);
#6329=AXIS2_PLACEMENT_3D('',#9003,#7181,#7182);
#6330=AXIS2_PLACEMENT_3D('',#9009,#7186,#7187);
#6331=AXIS2_PLACEMENT_3D('',#9012,#7190,#7191);
#6332=AXIS2_PLACEMENT_3D('',#9013,#7192,#7193);
#7004=DIRECTION('axis',(0.,0.,1.));
#7005=DIRECTION('refdir',(1.,0.,0.));
#7006=DIRECTION('center_axis',(1.,0.,0.));
#7007=DIRECTION('ref_axis',(0.,0.,-1.));
#7008=DIRECTION('center_axis',(1.,0.,0.));
#7009=DIRECTION('ref_axis',(0.,0.,-1.));
#7010=DIRECTION('',(1.,0.,0.));
#7011=DIRECTION('center_axis',(-1.,0.,0.));
#7012=DIRECTION('ref_axis',(0.,0.,-1.));
#7013=DIRECTION('center_axis',(1.,0.,0.));
#7014=DIRECTION('ref_axis',(0.,0.,-1.));
#7015=DIRECTION('center_axis',(1.,0.,0.));
#7016=DIRECTION('ref_axis',(0.,0.,-1.));
#7017=DIRECTION('',(1.,0.,0.));
#7018=DIRECTION('center_axis',(-1.,0.,0.));
#7019=DIRECTION('ref_axis',(0.,0.,-1.));
#7020=DIRECTION('center_axis',(1.,0.,0.));
#7021=DIRECTION('ref_axis',(0.,0.,-1.));
#7022=DIRECTION('center_axis',(1.,0.,0.));
#7023=DIRECTION('ref_axis',(0.,0.,-1.));
#7024=DIRECTION('',(1.,0.,0.));
#7025=DIRECTION('center_axis',(-1.,0.,0.));
#7026=DIRECTION('ref_axis',(0.,0.,-1.));
#7027=DIRECTION('center_axis',(1.,0.,0.));
#7028=DIRECTION('ref_axis',(0.,0.,-1.));
#7029=DIRECTION('center_axis',(1.,0.,0.));
#7030=DIRECTION('ref_axis',(0.,0.,-1.));
#7031=DIRECTION('',(1.,0.,0.));
#7032=DIRECTION('center_axis',(-1.,0.,0.));
#7033=DIRECTION('ref_axis',(0.,0.,-1.));
#7034=DIRECTION('center_axis',(1.,0.,0.));
#7035=DIRECTION('ref_axis',(0.,0.,-1.));
#7036=DIRECTION('center_axis',(1.,0.,0.));
#7037=DIRECTION('ref_axis',(0.,0.,-1.));
#7038=DIRECTION('',(1.,0.,0.));
#7039=DIRECTION('center_axis',(-1.,0.,0.));
#7040=DIRECTION('ref_axis',(0.,0.,-1.));
#7041=DIRECTION('center_axis',(1.,0.,0.));
#7042=DIRECTION('ref_axis',(0.,0.,-1.));
#7043=DIRECTION('center_axis',(1.,0.,0.));
#7044=DIRECTION('ref_axis',(0.,0.,-1.));
#7045=DIRECTION('',(-1.,0.,0.));
#7046=DIRECTION('center_axis',(-1.,0.,0.));
#7047=DIRECTION('ref_axis',(0.,0.,-1.));
#7048=DIRECTION('center_axis',(1.,0.,0.));
#7049=DIRECTION('ref_axis',(0.,0.,-1.));
#7050=DIRECTION('center_axis',(0.,0.,1.));
#7051=DIRECTION('ref_axis',(1.,0.,0.));
#7052=DIRECTION('center_axis',(0.,0.,1.));
#7053=DIRECTION('ref_axis',(1.,0.,0.));
#7054=DIRECTION('',(0.,0.,1.));
#7055=DIRECTION('center_axis',(0.,0.,-1.));
#7056=DIRECTION('ref_axis',(1.,0.,0.));
#7057=DIRECTION('center_axis',(0.,0.,1.));
#7058=DIRECTION('ref_axis',(1.,0.,0.));
#7059=DIRECTION('center_axis',(0.,0.,1.));
#7060=DIRECTION('ref_axis',(1.,0.,0.));
#7061=DIRECTION('center_axis',(0.,0.,1.));
#7062=DIRECTION('ref_axis',(1.,0.,0.));
#7063=DIRECTION('',(0.,0.,1.));
#7064=DIRECTION('center_axis',(0.,0.,-1.));
#7065=DIRECTION('ref_axis',(1.,0.,0.));
#7066=DIRECTION('center_axis',(0.,0.,-1.));
#7067=DIRECTION('ref_axis',(-1.,0.,0.));
#7068=DIRECTION('',(0.,-1.,0.));
#7069=DIRECTION('',(1.,0.,0.));
#7070=DIRECTION('',(0.,1.,0.));
#7071=DIRECTION('',(-1.,0.,0.));
#7072=DIRECTION('center_axis',(0.,0.,1.));
#7073=DIRECTION('ref_axis',(1.,0.,0.));
#7074=DIRECTION('',(0.,1.,0.));
#7075=DIRECTION('',(1.,0.,0.));
#7076=DIRECTION('',(0.,-1.,0.));
#7077=DIRECTION('',(-1.,0.,0.));
#7078=DIRECTION('center_axis',(0.,1.,0.));
#7079=DIRECTION('ref_axis',(0.,0.,1.));
#7080=DIRECTION('',(0.,0.,-1.));
#7081=DIRECTION('',(-1.,0.,0.));
#7082=DIRECTION('',(0.,0.,-1.));
#7083=DIRECTION('',(1.,0.,0.));
#7084=DIRECTION('',(0.,0.,-1.));
#7085=DIRECTION('center_axis',(0.,-1.,0.));
#7086=DIRECTION('ref_axis',(1.,0.,0.));
#7087=DIRECTION('center_axis',(0.,1.,0.));
#7088=DIRECTION('ref_axis',(-1.,0.,-1.22464679914735E-16));
#7089=DIRECTION('center_axis',(0.,1.,0.));
#7090=DIRECTION('ref_axis',(1.,0.,0.));
#7091=DIRECTION('center_axis',(1.,0.,0.));
#7092=DIRECTION('ref_axis',(0.,0.,-1.));
#7093=DIRECTION('',(0.,1.,0.));
#7094=DIRECTION('',(0.,0.,1.));
#7095=DIRECTION('center_axis',(0.,0.,-1.));
#7096=DIRECTION('ref_axis',(-1.,0.,0.));
#7097=DIRECTION('',(1.,0.,0.));
#7098=DIRECTION('',(0.,-1.,0.));
#7099=DIRECTION('',(0.,1.,0.));
#7100=DIRECTION('center_axis',(1.,0.,0.));
#7101=DIRECTION('ref_axis',(0.,0.,-1.));
#7102=DIRECTION('',(0.,0.,1.));
#7103=DIRECTION('center_axis',(0.,0.,1.));
#7104=DIRECTION('ref_axis',(1.,0.,0.));
#7105=DIRECTION('',(-1.,0.,0.));
#7106=DIRECTION('',(0.,1.,0.));
#7107=DIRECTION('center_axis',(0.,1.,0.));
#7108=DIRECTION('ref_axis',(1.,0.,0.));
#7109=DIRECTION('',(0.,0.,1.));
#7110=DIRECTION('center_axis',(0.,0.,1.));
#7111=DIRECTION('ref_axis',(1.,0.,0.));
#7112=DIRECTION('center_axis',(0.,0.,1.));
#7113=DIRECTION('ref_axis',(1.,0.,0.));
#7114=DIRECTION('',(0.,0.,1.));
#7115=DIRECTION('center_axis',(0.,0.,-1.));
#7116=DIRECTION('ref_axis',(1.,0.,0.));
#7117=DIRECTION('center_axis',(0.,0.,1.));
#7118=DIRECTION('ref_axis',(1.,0.,0.));
#7119=DIRECTION('center_axis',(0.,0.,1.));
#7120=DIRECTION('ref_axis',(1.,0.,0.));
#7121=DIRECTION('center_axis',(0.,0.,1.));
#7122=DIRECTION('ref_axis',(1.,0.,0.));
#7123=DIRECTION('',(0.,0.,1.));
#7124=DIRECTION('center_axis',(0.,0.,-1.));
#7125=DIRECTION('ref_axis',(1.,0.,0.));
#7126=DIRECTION('center_axis',(0.,0.,-1.));
#7127=DIRECTION('ref_axis',(-1.,0.,0.));
#7128=DIRECTION('',(0.,-1.,0.));
#7129=DIRECTION('',(1.,0.,0.));
#7130=DIRECTION('',(0.,1.,0.));
#7131=DIRECTION('',(-1.,0.,0.));
#7132=DIRECTION('center_axis',(0.,0.,1.));
#7133=DIRECTION('ref_axis',(1.,0.,0.));
#7134=DIRECTION('',(0.,1.,0.));
#7135=DIRECTION('',(1.,0.,0.));
#7136=DIRECTION('',(0.,-1.,0.));
#7137=DIRECTION('',(-1.,0.,0.));
#7138=DIRECTION('center_axis',(0.,1.,0.));
#7139=DIRECTION('ref_axis',(0.,0.,1.));
#7140=DIRECTION('',(0.,0.,-1.));
#7141=DIRECTION('',(-1.,0.,0.));
#7142=DIRECTION('',(0.,0.,-1.));
#7143=DIRECTION('',(1.,0.,0.));
#7144=DIRECTION('',(0.,0.,-1.));
#7145=DIRECTION('center_axis',(0.,-1.,0.));
#7146=DIRECTION('ref_axis',(1.,0.,0.));
#7147=DIRECTION('center_axis',(0.,1.,0.));
#7148=DIRECTION('ref_axis',(-1.,0.,-1.22464679914735E-16));
#7149=DIRECTION('center_axis',(0.,1.,0.));
#7150=DIRECTION('ref_axis',(1.,0.,0.));
#7151=DIRECTION('center_axis',(1.,0.,0.));
#7152=DIRECTION('ref_axis',(0.,0.,-1.));
#7153=DIRECTION('',(0.,1.,0.));
#7154=DIRECTION('',(0.,0.,1.));
#7155=DIRECTION('center_axis',(0.,0.,-1.));
#7156=DIRECTION('ref_axis',(-1.,0.,0.));
#7157=DIRECTION('',(1.,0.,0.));
#7158=DIRECTION('',(0.,-1.,0.));
#7159=DIRECTION('',(0.,1.,0.));
#7160=DIRECTION('center_axis',(1.,0.,0.));
#7161=DIRECTION('ref_axis',(0.,0.,-1.));
#7162=DIRECTION('',(0.,0.,1.));
#7163=DIRECTION('center_axis',(0.,0.,1.));
#7164=DIRECTION('ref_axis',(1.,0.,0.));
#7165=DIRECTION('',(-1.,0.,0.));
#7166=DIRECTION('',(0.,1.,0.));
#7167=DIRECTION('center_axis',(0.,1.,0.));
#7168=DIRECTION('ref_axis',(1.,0.,0.));
#7169=DIRECTION('',(0.,0.,1.));
#7170=DIRECTION('center_axis',(0.,1.,0.));
#7171=DIRECTION('ref_axis',(-1.,0.,0.));
#7172=DIRECTION('',(-1.,0.,0.));
#7173=DIRECTION('',(0.,0.,1.));
#7174=DIRECTION('',(-1.,0.,0.));
#7175=DIRECTION('',(0.,0.,1.));
#7176=DIRECTION('center_axis',(1.,0.,0.));
#7177=DIRECTION('ref_axis',(0.,1.,0.));
#7178=DIRECTION('',(0.,1.,0.));
#7179=DIRECTION('',(0.,1.,0.));
#7180=DIRECTION('',(0.,0.,1.));
#7181=DIRECTION('center_axis',(0.,-1.,0.));
#7182=DIRECTION('ref_axis',(1.,0.,0.));
#7183=DIRECTION('',(1.,0.,0.));
#7184=DIRECTION('',(1.,0.,0.));
#7185=DIRECTION('',(0.,0.,1.));
#7186=DIRECTION('center_axis',(-1.,0.,0.));
#7187=DIRECTION('ref_axis',(0.,-1.,0.));
#7188=DIRECTION('',(0.,-1.,0.));
#7189=DIRECTION('',(0.,-1.,0.));
#7190=DIRECTION('center_axis',(0.,0.,1.));
#7191=DIRECTION('ref_axis',(1.,0.,0.));
#7192=DIRECTION('center_axis',(0.,0.,1.));
#7193=DIRECTION('ref_axis',(1.,0.,0.));
#8826=CARTESIAN_POINT('',(0.,0.,0.));
#8827=CARTESIAN_POINT('Origin',(-4.5,8.5,3.));
#8828=CARTESIAN_POINT('',(-4.4,8.5,3.33));
#8829=CARTESIAN_POINT('Origin',(-4.4,8.5,3.));
#8830=CARTESIAN_POINT('',(-3.8,8.5,3.33));
#8831=CARTESIAN_POINT('',(-4.5,8.5,3.33));
#8832=CARTESIAN_POINT('Origin',(-3.8,8.5,3.));
#8833=CARTESIAN_POINT('Origin',(-4.5,-13.5,7.));
#8834=CARTESIAN_POINT('',(-4.4,-13.5,7.33));
#8835=CARTESIAN_POINT('Origin',(-4.4,-13.5,7.));
#8836=CARTESIAN_POINT('',(-3.8,-13.5,7.33));
#8837=CARTESIAN_POINT('',(-4.5,-13.5,7.33));
#8838=CARTESIAN_POINT('Origin',(-3.8,-13.5,7.));
#8839=CARTESIAN_POINT('Origin',(-4.5,-13.5,3.));
#8840=CARTESIAN_POINT('',(-4.4,-13.5,3.33));
#8841=CARTESIAN_POINT('Origin',(-4.4,-13.5,3.));
#8842=CARTESIAN_POINT('',(-3.8,-13.5,3.33));
#8843=CARTESIAN_POINT('',(-4.5,-13.5,3.33));
#8844=CARTESIAN_POINT('Origin',(-3.8,-13.5,3.));
#8845=CARTESIAN_POINT('Origin',(-4.5,8.5,7.));
#8846=CARTESIAN_POINT('',(-4.4,8.5,7.33));
#8847=CARTESIAN_POINT('Origin',(-4.4,8.5,7.));
#8848=CARTESIAN_POINT('',(-3.8,8.5,7.33));
#8849=CARTESIAN_POINT('',(-4.5,8.5,7.33));
#8850=CARTESIAN_POINT('Origin',(-3.8,8.5,7.));
#8851=CARTESIAN_POINT('Origin',(-4.5,-12.4,5.));
#8852=CARTESIAN_POINT('',(-4.4,-12.4,5.7));
#8853=CARTESIAN_POINT('Origin',(-4.4,-12.4,5.));
#8854=CARTESIAN_POINT('',(-3.5,-12.4,5.7));
#8855=CARTESIAN_POINT('',(-4.5,-12.4,5.7));
#8856=CARTESIAN_POINT('Origin',(-3.5,-12.4,5.));
#8857=CARTESIAN_POINT('Origin',(-3.8,-12.4,5.));
#8858=CARTESIAN_POINT('',(-3.5,-12.4,6.1));
#8859=CARTESIAN_POINT('Origin',(-3.5,-12.4,5.));
#8860=CARTESIAN_POINT('',(-3.8,-12.4,6.1));
#8861=CARTESIAN_POINT('',(-3.8,-12.4,6.1));
#8862=CARTESIAN_POINT('Origin',(-3.8,-12.4,5.));
#8863=CARTESIAN_POINT('Origin',(-3.5,-12.4,5.));
#8864=CARTESIAN_POINT('Origin',(2.2,7.,3.9));
#8865=CARTESIAN_POINT('',(1.95,7.,3.9));
#8866=CARTESIAN_POINT('Origin',(2.2,7.,3.9));
#8867=CARTESIAN_POINT('',(1.95,7.,4.95));
#8868=CARTESIAN_POINT('',(1.95,7.,3.9));
#8869=CARTESIAN_POINT('Origin',(2.2,7.,4.95));
#8870=CARTESIAN_POINT('Origin',(2.2,7.,3.9));
#8871=CARTESIAN_POINT('Origin',(2.2,7.,5.05));
#8872=CARTESIAN_POINT('',(1.87,7.,5.05));
#8873=CARTESIAN_POINT('Origin',(2.2,7.,5.05));
#8874=CARTESIAN_POINT('',(1.87,7.,7.));
#8875=CARTESIAN_POINT('',(1.87,7.,5.05));
#8876=CARTESIAN_POINT('Origin',(2.2,7.,7.));
#8877=CARTESIAN_POINT('Origin',(3.1,6.4,4.95));
#8878=CARTESIAN_POINT('',(3.,7.5,4.95));
#8879=CARTESIAN_POINT('',(3.,6.5,4.95));
#8880=CARTESIAN_POINT('',(3.,6.45,4.95));
#8881=CARTESIAN_POINT('',(1.50917195839308,7.5,4.95));
#8882=CARTESIAN_POINT('',(1.35,7.5,4.95));
#8883=CARTESIAN_POINT('',(1.50917195839308,6.5,4.95));
#8884=CARTESIAN_POINT('',(1.50917195839308,6.4,4.95));
#8885=CARTESIAN_POINT('',(1.35,6.5,4.95));
#8886=CARTESIAN_POINT('Origin',(0.,6.4,5.05));
#8887=CARTESIAN_POINT('',(3.,6.5,5.05));
#8888=CARTESIAN_POINT('',(3.,7.5,5.05));
#8889=CARTESIAN_POINT('',(3.,6.45,5.05));
#8890=CARTESIAN_POINT('',(1.50917195839308,6.5,5.05));
#8891=CARTESIAN_POINT('',(-0.2,6.5,5.05));
#8892=CARTESIAN_POINT('',(1.50917195839308,7.5,5.05));
#8893=CARTESIAN_POINT('',(1.50917195839308,6.4,5.05));
#8894=CARTESIAN_POINT('',(-0.2,7.5,5.05));
#8895=CARTESIAN_POINT('Origin',(-0.4,7.5,5.));
#8896=CARTESIAN_POINT('',(3.,7.5,3.));
#8897=CARTESIAN_POINT('',(3.,7.5,3.));
#8898=CARTESIAN_POINT('',(-3.8,7.5,3.));
#8899=CARTESIAN_POINT('',(-3.8,7.5,3.));
#8900=CARTESIAN_POINT('',(-3.8,7.5,7.));
#8901=CARTESIAN_POINT('',(-3.8,7.5,3.5));
#8902=CARTESIAN_POINT('',(3.,7.5,7.));
#8903=CARTESIAN_POINT('',(3.,7.5,7.));
#8904=CARTESIAN_POINT('',(3.,7.5,3.));
#8905=CARTESIAN_POINT('Origin',(0.,7.5,5.));
#8906=CARTESIAN_POINT('Origin',(0.,6.4,5.));
#8907=CARTESIAN_POINT('Origin',(0.,6.5,5.));
#8908=CARTESIAN_POINT('Origin',(3.,6.5,7.));
#8909=CARTESIAN_POINT('',(3.,6.5,7.));
#8910=CARTESIAN_POINT('',(3.,6.5,7.));
#8911=CARTESIAN_POINT('',(3.,6.5,3.));
#8912=CARTESIAN_POINT('Origin',(3.,6.5,3.));
#8913=CARTESIAN_POINT('',(-3.8,6.5,3.));
#8914=CARTESIAN_POINT('',(3.,6.5,3.));
#8915=CARTESIAN_POINT('',(-3.8,6.5,3.));
#8916=CARTESIAN_POINT('',(-3.8,-4.,3.));
#8917=CARTESIAN_POINT('',(3.,6.5,3.));
#8918=CARTESIAN_POINT('Origin',(3.,6.5,7.));
#8919=CARTESIAN_POINT('',(3.,6.5,3.));
#8920=CARTESIAN_POINT('Origin',(-3.8,6.5,7.));
#8921=CARTESIAN_POINT('',(-3.8,6.5,7.));
#8922=CARTESIAN_POINT('',(3.,6.5,7.));
#8923=CARTESIAN_POINT('',(-3.8,-4.,7.));
#8924=CARTESIAN_POINT('Origin',(-0.4,6.5,5.));
#8925=CARTESIAN_POINT('',(-3.8,6.5,3.5));
#8926=CARTESIAN_POINT('Origin',(2.2,-7.,3.9));
#8927=CARTESIAN_POINT('',(1.95,-7.,3.9));
#8928=CARTESIAN_POINT('Origin',(2.2,-7.,3.9));
#8929=CARTESIAN_POINT('',(1.95,-7.,4.95));
#8930=CARTESIAN_POINT('',(1.95,-7.,3.9));
#8931=CARTESIAN_POINT('Origin',(2.2,-7.,4.95));
#8932=CARTESIAN_POINT('Origin',(2.2,-7.,3.9));
#8933=CARTESIAN_POINT('Origin',(2.2,-7.,5.05));
#8934=CARTESIAN_POINT('',(1.87,-7.,5.05));
#8935=CARTESIAN_POINT('Origin',(2.2,-7.,5.05));
#8936=CARTESIAN_POINT('',(1.87,-7.,7.));
#8937=CARTESIAN_POINT('',(1.87,-7.,5.05));
#8938=CARTESIAN_POINT('Origin',(2.2,-7.,7.));
#8939=CARTESIAN_POINT('Origin',(3.1,-7.6,4.95));
#8940=CARTESIAN_POINT('',(3.,-6.5,4.95));
#8941=CARTESIAN_POINT('',(3.,-7.5,4.95));
#8942=CARTESIAN_POINT('',(3.,-7.55,4.95));
#8943=CARTESIAN_POINT('',(1.50917195839308,-6.5,4.95));
#8944=CARTESIAN_POINT('',(1.35,-6.5,4.95));
#8945=CARTESIAN_POINT('',(1.50917195839308,-7.5,4.95));
#8946=CARTESIAN_POINT('',(1.50917195839308,-7.6,4.95));
#8947=CARTESIAN_POINT('',(1.35,-7.5,4.95));
#8948=CARTESIAN_POINT('Origin',(0.,-7.6,5.05));
#8949=CARTESIAN_POINT('',(3.,-7.5,5.05));
#8950=CARTESIAN_POINT('',(3.,-6.5,5.05));
#8951=CARTESIAN_POINT('',(3.,-7.55,5.05));
#8952=CARTESIAN_POINT('',(1.50917195839308,-7.5,5.05));
#8953=CARTESIAN_POINT('',(-0.2,-7.5,5.05));
#8954=CARTESIAN_POINT('',(1.50917195839308,-6.5,5.05));
#8955=CARTESIAN_POINT('',(1.50917195839308,-7.6,5.05));
#8956=CARTESIAN_POINT('',(-0.2,-6.5,5.05));
#8957=CARTESIAN_POINT('Origin',(-0.4,-6.5,5.));
#8958=CARTESIAN_POINT('',(3.,-6.5,3.));
#8959=CARTESIAN_POINT('',(3.,-6.5,3.));
#8960=CARTESIAN_POINT('',(-3.8,-6.5,3.));
#8961=CARTESIAN_POINT('',(-3.8,-6.5,3.));
#8962=CARTESIAN_POINT('',(-3.8,-6.5,7.));
#8963=CARTESIAN_POINT('',(-3.8,-6.5,3.5));
#8964=CARTESIAN_POINT('',(3.,-6.5,7.));
#8965=CARTESIAN_POINT('',(3.,-6.5,7.));
#8966=CARTESIAN_POINT('',(3.,-6.5,3.));
#8967=CARTESIAN_POINT('Origin',(0.,-6.5,5.));
#8968=CARTESIAN_POINT('Origin',(0.,-7.6,5.));
#8969=CARTESIAN_POINT('Origin',(0.,-7.5,5.));
#8970=CARTESIAN_POINT('Origin',(3.,-7.5,7.));
#8971=CARTESIAN_POINT('',(3.,-7.5,7.));
#8972=CARTESIAN_POINT('',(3.,-7.5,7.));
#8973=CARTESIAN_POINT('',(3.,-7.5,3.));
#8974=CARTESIAN_POINT('Origin',(3.,-7.5,3.));
#8975=CARTESIAN_POINT('',(-3.8,-7.5,3.));
#8976=CARTESIAN_POINT('',(3.,-7.5,3.));
#8977=CARTESIAN_POINT('',(-3.8,-7.5,3.));
#8978=CARTESIAN_POINT('',(-3.8,-11.,3.));
#8979=CARTESIAN_POINT('',(3.,-7.5,3.));
#8980=CARTESIAN_POINT('Origin',(3.,-7.5,7.));
#8981=CARTESIAN_POINT('',(3.,-7.5,3.));
#8982=CARTESIAN_POINT('Origin',(-3.8,-7.5,7.));
#8983=CARTESIAN_POINT('',(-3.8,-7.5,7.));
#8984=CARTESIAN_POINT('',(3.,-7.5,7.));
#8985=CARTESIAN_POINT('',(-3.8,-11.,7.));
#8986=CARTESIAN_POINT('Origin',(-0.4,-7.5,5.));
#8987=CARTESIAN_POINT('',(-3.8,-7.5,3.5));
#8988=CARTESIAN_POINT('Origin',(-3.8,9.5,2.));
#8989=CARTESIAN_POINT('',(-3.8,9.5,2.));
#8990=CARTESIAN_POINT('',(-4.4,9.5,2.));
#8991=CARTESIAN_POINT('',(-3.8,9.5,2.));
#8992=CARTESIAN_POINT('',(-4.4,9.5,8.));
#8993=CARTESIAN_POINT('',(-4.4,9.5,2.));
#8994=CARTESIAN_POINT('',(-3.8,9.5,8.));
#8995=CARTESIAN_POINT('',(-3.8,9.5,8.));
#8996=CARTESIAN_POINT('',(-3.8,9.5,2.));
#8997=CARTESIAN_POINT('Origin',(-3.8,-14.5,2.));
#8998=CARTESIAN_POINT('',(-3.8,-14.5,2.));
#8999=CARTESIAN_POINT('',(-3.8,-14.5,2.));
#9000=CARTESIAN_POINT('',(-3.8,-14.5,8.));
#9001=CARTESIAN_POINT('',(-3.8,-14.5,8.));
#9002=CARTESIAN_POINT('',(-3.8,-14.5,2.));
#9003=CARTESIAN_POINT('Origin',(-4.4,-14.5,2.));
#9004=CARTESIAN_POINT('',(-4.4,-14.5,2.));
#9005=CARTESIAN_POINT('',(-4.4,-14.5,2.));
#9006=CARTESIAN_POINT('',(-4.4,-14.5,8.));
#9007=CARTESIAN_POINT('',(-4.4,-14.5,8.));
#9008=CARTESIAN_POINT('',(-4.4,-14.5,2.));
#9009=CARTESIAN_POINT('Origin',(-4.4,9.5,2.));
#9010=CARTESIAN_POINT('',(-4.4,9.5,2.));
#9011=CARTESIAN_POINT('',(-4.4,9.5,8.));
#9012=CARTESIAN_POINT('Origin',(-4.1,-2.5,8.));
#9013=CARTESIAN_POINT('Origin',(-4.1,-2.5,2.));
#10456=UNCERTAINTY_MEASURE_WITH_UNIT(LENGTH_MEASURE(0.001),#10518,
'DISTANCE_ACCURACY_VALUE',
'Maximum model space distance between geometric entities at asserted c
onnectivities');
#10484=UNCERTAINTY_MEASURE_WITH_UNIT(LENGTH_MEASURE(0.001),#10518,
'DISTANCE_ACCURACY_VALUE',
'Maximum model space distance between geometric entities at asserted c
onnectivities');
#10489=(
GEOMETRIC_REPRESENTATION_CONTEXT(3)
GLOBAL_UNCERTAINTY_ASSIGNED_CONTEXT((#10456))
GLOBAL_UNIT_ASSIGNED_CONTEXT((#10518,#10520,#10521))
REPRESENTATION_CONTEXT('','3D')
);
#10517=(
GEOMETRIC_REPRESENTATION_CONTEXT(3)
GLOBAL_UNCERTAINTY_ASSIGNED_CONTEXT((#10484))
GLOBAL_UNIT_ASSIGNED_CONTEXT((#10518,#10520,#10521))
REPRESENTATION_CONTEXT('','3D')
);
#10518=(
LENGTH_UNIT()
NAMED_UNIT(*)
SI_UNIT(.CENTI.,.METRE.)
);
#10520=(
NAMED_UNIT(*)
PLANE_ANGLE_UNIT()
SI_UNIT($,.RADIAN.)
);
#10521=(
NAMED_UNIT(*)
SI_UNIT($,.STERADIAN.)
SOLID_ANGLE_UNIT()
);
#10526=SHAPE_DEFINITION_REPRESENTATION(#10558,#10645);
#10558=PRODUCT_DEFINITION_SHAPE('',$,#10678);
#10645=SHAPE_REPRESENTATION('',(#6271),#10489);
#10673=PRODUCT_DEFINITION_CONTEXT('part definition',#10771,'design');
#10678=PRODUCT_DEFINITION('Wall bracket','Wall bracket',#10710,#10673);
#10710=PRODUCT_DEFINITION_FORMATION('',$,#10777);
#10771=APPLICATION_CONTEXT(
'Core Data for Automotive Mechanical Design Process');
#10772=PRODUCT_CONTEXT('part definition',#10771,'mechanical');
#10777=PRODUCT('Wall bracket','Wall bracket','Wall bracket',(#10772));
#10847=COLOUR_RGB('Dark Blue',0.08,0.2,0.34);
#10848=FILL_AREA_STYLE_COLOUR('',#10847);
#10849=FILL_AREA_STYLE('',(#10848));
#10850=SURFACE_STYLE_FILL_AREA(#10849);
#10851=SURFACE_SIDE_STYLE('',(#10850));
#10852=SURFACE_STYLE_USAGE(.BOTH.,#10851);
#10853=PRESENTATION_STYLE_ASSIGNMENT((#10852));
ENDSEC;
END-ISO-10303-21;
